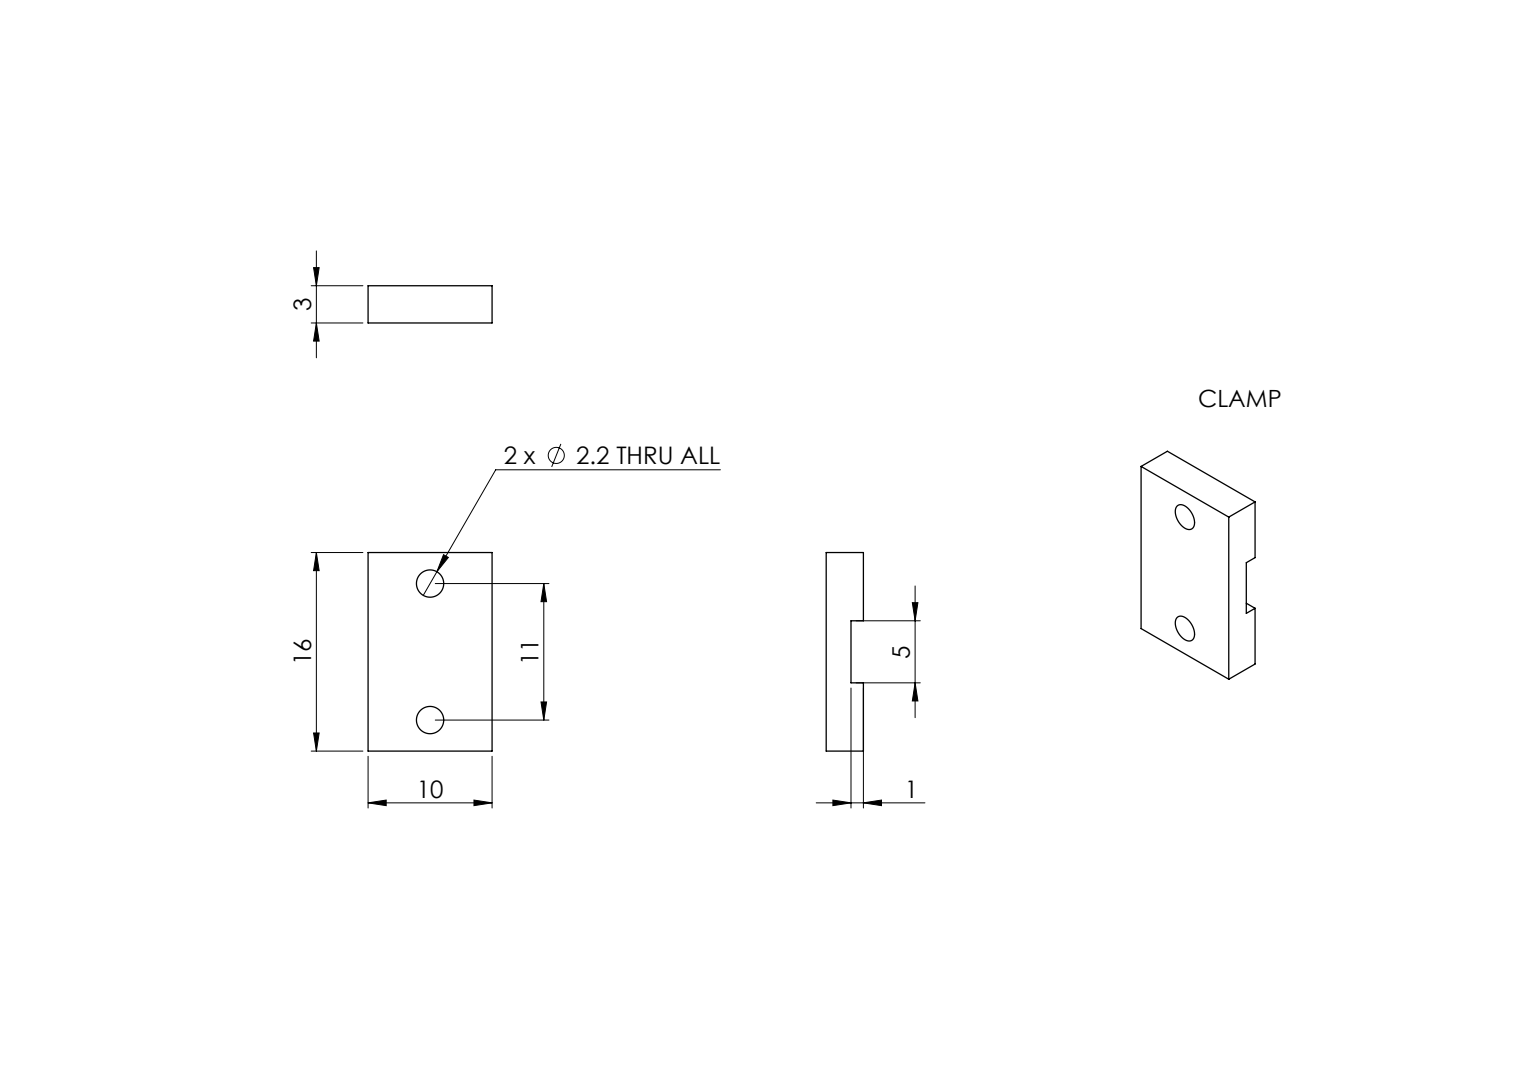
ISO-10303-21;
HEADER;
FILE_DESCRIPTION (('STEP AP214'),
    '1' );
FILE_NAME ('clamp.step',
    '2026-10-27T04:40:18',
    ( '' ),
    ( '' ),
    'SwSTEP 2.0',
    'SolidWorks 2026',
    '' );
FILE_SCHEMA (( 'AUTOMOTIVE_DESIGN' ));
ENDSEC;

DATA;
#33=ORIENTED_EDGE ( 'NONE', *, *, #3045, .T. ) ;
#39=ADVANCED_FACE ( 'NONE', ( #10062, #3972, #586 ), #1625, .F. ) ;
#93=ORIENTED_EDGE ( 'NONE', *, *, #6556, .F. ) ;
#105=CARTESIAN_POINT ( 'NONE',  ( 140.0000000000000284, 8.000000000000000000, 3.000000000000000000 ) ) ;
#116=PLANE ( 'NONE',  #5116 ) ;
#128=ORIENTED_EDGE ( 'NONE', *, *, #1993, .F. ) ;
#135=CARTESIAN_POINT ( 'NONE',  ( -105.0000000000000000, 2.500000000000000000, 4.000000000000000000 ) ) ;
#148=VECTOR ( 'NONE', #1244, 1000.000000000000000 ) ;
#149=ORIENTED_EDGE ( 'NONE', *, *, #772, .F. ) ;
#199=EDGE_LOOP ( 'NONE', ( #1282, #1739, #251, #2267 ) ) ;
#206=CLOSED_SHELL ( 'NONE', ( #8673, #5883, #7933, #4871, #589, #6929, #9618, #1051, #39, #10363, #9693, #7084, #2486, #5406 ) ) ;
#212=AXIS2_PLACEMENT_3D ( 'NONE', #5369, #8063, #3772 ) ;
#233=APPLICATION_CONTEXT ( 'automotive_design' ) ;
#234=VECTOR ( 'NONE', #2072, 1000.000000000000000 ) ;
#244=LINE ( 'NONE', #5283, #6807 ) ;
#251=ORIENTED_EDGE ( 'NONE', *, *, #8511, .F. ) ;
#342=DIRECTION ( 'NONE',  ( 0.000000000000000000, 0.000000000000000000, 1.000000000000000000 ) ) ;
#380=LINE ( 'NONE', #7160, #836 ) ;
#399=PRODUCT_DEFINITION_CONTEXT ( 'detailed design', #1660, 'design' ) ;
#402=CIRCLE ( 'NONE', #212, 1.099999999999989875 ) ;
#445=EDGE_CURVE ( 'NONE', #6076, #9310, #10674, .T. ) ;
#450=ORIENTED_EDGE ( 'NONE', *, *, #772, .T. ) ;
#469=DIRECTION ( 'NONE',  ( 1.000000000000000000, 0.000000000000000000, 0.000000000000000000 ) ) ;
#487=LINE ( 'NONE', #3873, #692 ) ;
#502=ORIENTED_EDGE ( 'NONE', *, *, #6812, .F. ) ;
#511=CARTESIAN_POINT ( 'NONE',  ( 150.0000000000000000, -2.500000000000000444, 6.000000000000000000 ) ) ;
#578=ORIENTED_EDGE ( 'NONE', *, *, #2504, .T. ) ;
#586=FACE_OUTER_BOUND ( 'NONE', #5446, .T. ) ;
#589=ADVANCED_FACE ( 'NONE', ( #5826, #10002 ), #5614, .T. ) ;
#591=VECTOR ( 'NONE', #8546, 1000.000000000000000 ) ;
#651=ORIENTED_EDGE ( 'NONE', *, *, #6556, .T. ) ;
#669=ORIENTED_EDGE ( 'NONE', *, *, #6090, .F. ) ;
#692=VECTOR ( 'NONE', #10647, 1000.000000000000000 ) ;
#702=MECHANICAL_DESIGN_GEOMETRIC_PRESENTATION_REPRESENTATION('',(#1232),#9754);
#743=VECTOR ( 'NONE', #342, 1000.000000000000000 ) ;
#764=CIRCLE ( 'NONE', #5367, 1.099999999999989875 ) ;
#772=EDGE_CURVE ( 'NONE', #7557, #5975, #6044, .T. ) ;
#798=ORIENTED_EDGE ( 'NONE', *, *, #2162, .T. ) ;
#831=DIRECTION ( 'NONE',  ( -0.000000000000000000, 1.000000000000000000, 0.000000000000000000 ) ) ;
#836=VECTOR ( 'NONE', #5537, 1000.000000000000000 ) ;
#847=VERTEX_POINT ( 'NONE', #1713 ) ;
#928=EDGE_CURVE ( 'NONE', #847, #6070, #402, .T. ) ;
#944=CYLINDRICAL_SURFACE ( 'NONE', #4058, 1.099999999999989875 ) ;
#953=ORIENTED_EDGE ( 'NONE', *, *, #8718, .T. ) ;
#970=SURFACE_STYLE_USAGE ( .BOTH. , #1755 ) ;
#979=DIRECTION ( 'NONE',  ( 0.000000000000000000, -0.000000000000000000, -1.000000000000000000 ) ) ;
#983=ORIENTED_EDGE ( 'NONE', *, *, #2088, .F. ) ;
#999=DIRECTION ( 'NONE',  ( -1.000000000000000000, 0.000000000000000000, -0.000000000000000000 ) ) ;
#1017=CYLINDRICAL_SURFACE ( 'NONE', #3505, 1.099999999999989875 ) ;
#1024=FACE_OUTER_BOUND ( 'NONE', #3434, .T. ) ;
#1045=VECTOR ( 'NONE', #1236, 1000.000000000000000 ) ;
#1051=ADVANCED_FACE ( 'NONE', ( #3001 ), #6391, .F. ) ;
#1098=DIRECTION ( 'NONE',  ( 0.000000000000000000, 1.000000000000000000, 0.000000000000000000 ) ) ;
#1126=FACE_OUTER_BOUND ( 'NONE', #4388, .T. ) ;
#1133=ORIENTED_EDGE ( 'NONE', *, *, #1752, .T. ) ;
#1136=VERTEX_POINT ( 'NONE', #5803 ) ;
#1154=EDGE_CURVE ( 'NONE', #5040, #5356, #5860, .T. ) ;
#1226=FACE_OUTER_BOUND ( 'NONE', #5077, .T. ) ;
#1232=STYLED_ITEM ( 'NONE', ( #2645 ), #7886 ) ;
#1236=DIRECTION ( 'NONE',  ( -0.000000000000000000, -0.000000000000000000, 1.000000000000000000 ) ) ;
#1244=DIRECTION ( 'NONE',  ( -1.000000000000000000, 0.000000000000000000, 0.000000000000000000 ) ) ;
#1282=ORIENTED_EDGE ( 'NONE', *, *, #6378, .T. ) ;
#1324=VECTOR ( 'NONE', #9947, 1000.000000000000000 ) ;
#1328=CARTESIAN_POINT ( 'NONE',  ( 143.9000000000000341, 5.500000000000000000, 6.000000000000000000 ) ) ;
#1398=VECTOR ( 'NONE', #3895, 1000.000000000000000 ) ;
#1472=ORIENTED_EDGE ( 'NONE', *, *, #9040, .T. ) ;
#1505=EDGE_LOOP ( 'NONE', ( #10466, #4149, #3036, #8916 ) ) ;
#1508=ORIENTED_EDGE ( 'NONE', *, *, #1752, .F. ) ;
#1522=ORIENTED_EDGE ( 'NONE', *, *, #1154, .F. ) ;
#1556=PRODUCT_DEFINITION_SHAPE ( 'NONE', 'NONE',  #1620 ) ;
#1557=ORIENTED_EDGE ( 'NONE', *, *, #6848, .T. ) ;
#1560=LINE ( 'NONE', #8344, #5022 ) ;
#1594=AXIS2_PLACEMENT_3D ( 'NONE', #1609, #8605, #4362 ) ;
#1609=CARTESIAN_POINT ( 'NONE',  ( 145.0000000000000284, 5.500000000000000000, 6.000000000000000000 ) ) ;
#1620=PRODUCT_DEFINITION ( 'UNKNOWN', '', #6403, #399 ) ;
#1625=PLANE ( 'NONE',  #9971 ) ;
#1648=VERTEX_POINT ( 'NONE', #5161 ) ;
#1660=APPLICATION_CONTEXT ( 'automotive_design' ) ;
#1663=FACE_OUTER_BOUND ( 'NONE', #6726, .T. ) ;
#1706=DIRECTION ( 'NONE',  ( 1.000000000000000000, 0.000000000000000000, 0.000000000000000000 ) ) ;
#1713=CARTESIAN_POINT ( 'NONE',  ( 143.9000000000000341, -5.500000000000000000, 6.000000000000000000 ) ) ;
#1739=ORIENTED_EDGE ( 'NONE', *, *, #7365, .F. ) ;
#1752=EDGE_CURVE ( 'NONE', #1136, #10538, #8935, .T. ) ;
#1755=SURFACE_SIDE_STYLE ('',( #5970 ) ) ;
#1816=DIRECTION ( 'NONE',  ( -0.000000000000000000, -0.000000000000000000, 1.000000000000000000 ) ) ;
#1846=CARTESIAN_POINT ( 'NONE',  ( 146.0999999999999943, -5.500000000000000000, 6.000000000000000000 ) ) ;
#1877=EDGE_CURVE ( 'NONE', #1648, #10538, #7962, .T. ) ;
#1898=ORIENTED_EDGE ( 'NONE', *, *, #3692, .T. ) ;
#1908=STYLED_ITEM('',(#11006),#8465);
#1929=EDGE_CURVE ( 'NONE', #10524, #8381, #2909, .T. ) ;
#1939=EDGE_LOOP ( 'NONE', ( #6034, #3156, #1522, #2323 ) ) ;
#1965=CARTESIAN_POINT ( 'NONE',  ( 150.0000000000000000, 8.000000000000000000, 3.000000000000000000 ) ) ;
#1981=FILL_AREA_STYLE_COLOUR ( '', #9214 ) ;
#1993=EDGE_CURVE ( 'NONE', #10287, #2286, #7346, .T. ) ;
#2045=DIRECTION ( 'NONE',  ( -0.000000000000000000, -1.000000000000000000, -0.000000000000000000 ) ) ;
#2055=CARTESIAN_POINT ( 'NONE',  ( 150.0000000000000000, -8.000000000000000000, 6.000000000000000000 ) ) ;
#2072=DIRECTION ( 'NONE',  ( 1.000000000000000000, -0.000000000000000000, 0.000000000000000000 ) ) ;
#2084=DIRECTION ( 'NONE',  ( -0.000000000000000000, -0.000000000000000000, 1.000000000000000000 ) ) ;
#2088=EDGE_CURVE ( 'NONE', #5975, #8381, #10227, .T. ) ;
#2098=ORIENTED_EDGE ( 'NONE', *, *, #4861, .F. ) ;
#2099=( GEOMETRIC_REPRESENTATION_CONTEXT ( 3 ) GLOBAL_UNCERTAINTY_ASSIGNED_CONTEXT ( ( #7955 ) ) GLOBAL_UNIT_ASSIGNED_CONTEXT ( ( #3880, #2217, #6383 ) ) REPRESENTATION_CONTEXT ( 'NONE', 'WORKASPACE' ) );
#2118=DIRECTION ( 'NONE',  ( -0.000000000000000000, -0.000000000000000000, 1.000000000000000000 ) ) ;
#2129=CARTESIAN_POINT ( 'NONE',  ( 146.0999999999999943, 5.500000000000000000, 6.000000000000000000 ) ) ;
#2130=DIRECTION ( 'NONE',  ( -0.000000000000000000, -0.000000000000000000, 1.000000000000000000 ) ) ;
#2144=AXIS2_PLACEMENT_3D ( 'NONE', #4502, #10617, #3015 ) ;
#2162=EDGE_CURVE ( 'NONE', #9310, #7235, #244, .T. ) ;
#2217=( NAMED_UNIT ( * ) PLANE_ANGLE_UNIT ( ) SI_UNIT ( $, .RADIAN. ) );
#2267=ORIENTED_EDGE ( 'NONE', *, *, #6909, .T. ) ;
#2286=VERTEX_POINT ( 'NONE', #10633 ) ;
#2298=EDGE_CURVE ( 'NONE', #9621, #5032, #764, .T. ) ;
#2307=AXIS2_PLACEMENT_3D ( 'NONE', #5193, #3646, #1706 ) ;
#2319=ORIENTED_EDGE ( 'NONE', *, *, #2298, .F. ) ;
#2323=ORIENTED_EDGE ( 'NONE', *, *, #6378, .F. ) ;
#2368=VECTOR ( 'NONE', #2130, 1000.000000000000000 ) ;
#2383=CARTESIAN_POINT ( 'NONE',  ( 0.000000000000000000, 0.000000000000000000, 3.000000000000000000 ) ) ;
#2412=DIRECTION ( 'NONE',  ( -0.000000000000000000, -1.000000000000000000, -0.000000000000000000 ) ) ;
#2439=DIRECTION ( 'NONE',  ( 0.000000000000000000, 1.000000000000000000, 0.000000000000000000 ) ) ;
#2441=DIRECTION ( 'NONE',  ( 1.000000000000000000, 0.000000000000000000, 0.000000000000000000 ) ) ;
#2464=ORIENTED_EDGE ( 'NONE', *, *, #4239, .T. ) ;
#2466=EDGE_CURVE ( 'NONE', #6070, #847, #10155, .T. ) ;
#2486=ADVANCED_FACE ( 'NONE', ( #5941 ), #6580, .F. ) ;
#2488=ORIENTED_EDGE ( 'NONE', *, *, #6301, .T. ) ;
#2494=CARTESIAN_POINT ( 'NONE',  ( 150.0000000000000000, -8.000000000000000000, 6.000000000000000000 ) ) ;
#2504=EDGE_CURVE ( 'NONE', #10287, #7557, #1560, .T. ) ;
#2512=FACE_BOUND ( 'NONE', #4343, .T. ) ;
#2518=LINE ( 'NONE', #6693, #6429 ) ;
#2549=ORIENTED_EDGE ( 'NONE', *, *, #2298, .T. ) ;
#2566=DIRECTION ( 'NONE',  ( 1.000000000000000000, 0.000000000000000000, 0.000000000000000000 ) ) ;
#2589=CARTESIAN_POINT ( 'NONE',  ( 140.0000000000000284, 8.000000000000000000, 3.000000000000000000 ) ) ;
#2645=PRESENTATION_STYLE_ASSIGNMENT (( #970 ) ) ;
#2715=VECTOR ( 'NONE', #6517, 1000.000000000000000 ) ;
#2751=DIRECTION ( 'NONE',  ( 1.000000000000000000, 0.000000000000000000, 0.000000000000000000 ) ) ;
#2842=CARTESIAN_POINT ( 'NONE',  ( 140.0000000000000568, 2.500000000000000000, 4.000000000000000000 ) ) ;
#2909=LINE ( 'NONE', #6296, #234 ) ;
#2954=CARTESIAN_POINT ( 'NONE',  ( 140.0000000000000284, 2.500000000000000000, 3.000000000000000000 ) ) ;
#2963=LINE ( 'NONE', #2129, #1045 ) ;
#3001=FACE_OUTER_BOUND ( 'NONE', #5813, .T. ) ;
#3003=CARTESIAN_POINT ( 'NONE',  ( 150.0000000000000000, -8.000000000000000000, 6.000000000000000000 ) ) ;
#3015=DIRECTION ( 'NONE',  ( 0.000000000000000000, -0.000000000000000000, 1.000000000000000000 ) ) ;
#3036=ORIENTED_EDGE ( 'NONE', *, *, #7473, .T. ) ;
#3045=EDGE_CURVE ( 'NONE', #9310, #5427, #7645, .T. ) ;
#3121=CARTESIAN_POINT ( 'NONE',  ( 140.0000000000000284, -8.000000000000000000, 6.000000000000000000 ) ) ;
#3156=ORIENTED_EDGE ( 'NONE', *, *, #4861, .T. ) ;
#3176=CARTESIAN_POINT ( 'NONE',  ( 150.0000000000000000, 8.000000000000000000, 6.000000000000000000 ) ) ;
#3217=CARTESIAN_POINT ( 'NONE',  ( 150.0000000000000284, -2.500000000000000000, 4.000000000000000000 ) ) ;
#3319=PLANE ( 'NONE',  #10244 ) ;
#3338=CARTESIAN_POINT ( 'NONE',  ( 0.000000000000000000, 0.000000000000000000, 3.000000000000000000 ) ) ;
#3365=DIRECTION ( 'NONE',  ( 1.000000000000000000, 0.000000000000000000, 0.000000000000000000 ) ) ;
#3409=CARTESIAN_POINT ( 'NONE',  ( 140.0000000000000284, -8.000000000000000000, 3.000000000000000000 ) ) ;
#3427=AXIS2_PLACEMENT_3D ( 'NONE', #5834, #8445, #10785 ) ;
#3434=EDGE_LOOP ( 'NONE', ( #798, #10069, #3716, #5140 ) ) ;
#3469=( LENGTH_UNIT ( ) NAMED_UNIT ( * ) SI_UNIT ( .MILLI., .METRE. ) );
#3474=DIRECTION ( 'NONE',  ( -1.000000000000000000, -0.000000000000000000, -0.000000000000000000 ) ) ;
#3505=AXIS2_PLACEMENT_3D ( 'NONE', #5175, #5124, #2751 ) ;
#3518=AXIS2_PLACEMENT_3D ( 'NONE', #8801, #469, #10626 ) ;
#3554=CARTESIAN_POINT ( 'NONE',  ( 150.0000000000000000, 2.500000000000000000, 3.000000000000000000 ) ) ;
#3557=ORIENTED_EDGE ( 'NONE', *, *, #1877, .F. ) ;
#3588=VECTOR ( 'NONE', #2412, 1000.000000000000000 ) ;
#3597=CARTESIAN_POINT ( 'NONE',  ( 140.0000000000000284, -8.000000000000000000, 6.000000000000000000 ) ) ;
#3634=VERTEX_POINT ( 'NONE', #4108 ) ;
#3646=DIRECTION ( 'NONE',  ( 0.000000000000000000, 0.000000000000000000, 1.000000000000000000 ) ) ;
#3670=CARTESIAN_POINT ( 'NONE',  ( 145.0000000000000284, 5.500000000000000000, 6.000000000000000000 ) ) ;
#3690=ORIENTED_EDGE ( 'NONE', *, *, #928, .F. ) ;
#3692=EDGE_CURVE ( 'NONE', #10524, #3634, #7507, .T. ) ;
#3709=VECTOR ( 'NONE', #5631, 1000.000000000000000 ) ;
#3716=ORIENTED_EDGE ( 'NONE', *, *, #5091, .T. ) ;
#3764=EDGE_CURVE ( 'NONE', #7557, #4954, #5831, .T. ) ;
#3768=AXIS2_PLACEMENT_3D ( 'NONE', #3597, #1098, #6158 ) ;
#3772=DIRECTION ( 'NONE',  ( 1.000000000000000000, 0.000000000000000000, 0.000000000000000000 ) ) ;
#3819=SHAPE_REPRESENTATION_RELATIONSHIP ( 'NONE' , 'NONE' ,  #10405, #7886 ) ;
#3832=ORIENTED_EDGE ( 'NONE', *, *, #928, .T. ) ;
#3873=CARTESIAN_POINT ( 'NONE',  ( 150.0000000000000000, -8.000000000000000000, 3.000000000000000000 ) ) ;
#3876=ORIENTED_EDGE ( 'NONE', *, *, #7132, .T. ) ;
#3880=( LENGTH_UNIT ( ) NAMED_UNIT ( * ) SI_UNIT ( .MILLI., .METRE. ) );
#3895=DIRECTION ( 'NONE',  ( 0.000000000000000000, 0.000000000000000000, -1.000000000000000000 ) ) ;
#3903=LINE ( 'NONE', #7294, #6212 ) ;
#3972=FACE_BOUND ( 'NONE', #5458, .T. ) ;
#4007=DIRECTION ( 'NONE',  ( 0.000000000000000000, 0.000000000000000000, 1.000000000000000000 ) ) ;
#4058=AXIS2_PLACEMENT_3D ( 'NONE', #9334, #7732, #8404 ) ;
#4071=VECTOR ( 'NONE', #2045, 1000.000000000000000 ) ;
#4095=DIRECTION ( 'NONE',  ( -1.000000000000000000, 0.000000000000000000, 0.000000000000000000 ) ) ;
#4108=CARTESIAN_POINT ( 'NONE',  ( 140.0000000000000568, -2.500000000000000000, 4.000000000000000000 ) ) ;
#4132=EDGE_LOOP ( 'NONE', ( #5405, #2319, #1557, #4656 ) ) ;
#4149=ORIENTED_EDGE ( 'NONE', *, *, #1877, .T. ) ;
#4228=ORIENTED_EDGE ( 'NONE', *, *, #5091, .F. ) ;
#4239=EDGE_CURVE ( 'NONE', #5427, #5356, #9469, .T. ) ;
#4246=DIRECTION ( 'NONE',  ( -0.000000000000000000, -0.000000000000000000, 1.000000000000000000 ) ) ;
#4272=CARTESIAN_POINT ( 'NONE',  ( 150.0000000000000000, 8.000000000000000000, 6.000000000000000000 ) ) ;
#4284=DIRECTION ( 'NONE',  ( 0.000000000000000000, -1.000000000000000000, 0.000000000000000000 ) ) ;
#4327=DIRECTION ( 'NONE',  ( -0.000000000000000000, -0.000000000000000000, -1.000000000000000000 ) ) ;
#4343=EDGE_LOOP ( 'NONE', ( #2549, #2488 ) ) ;
#4346=( LENGTH_UNIT ( ) NAMED_UNIT ( * ) SI_UNIT ( .MILLI., .METRE. ) );
#4362=DIRECTION ( 'NONE',  ( 1.000000000000000000, 0.000000000000000000, 0.000000000000000000 ) ) ;
#4369=CARTESIAN_POINT ( 'NONE',  ( 140.0000000000000284, -8.000000000000000000, 4.000000000000000000 ) ) ;
#4388=EDGE_LOOP ( 'NONE', ( #4659, #4228, #5013, #651, #128, #502, #8779, #5188 ) ) ;
#4396=AXIS2_PLACEMENT_3D ( 'NONE', #4668, #4825, #8181 ) ;
#4414=LINE ( 'NONE', #5357, #4071 ) ;
#4472=VECTOR ( 'NONE', #4007, 1000.000000000000000 ) ;
#4480=EDGE_LOOP ( 'NONE', ( #6392, #5597, #10932, #8542, #450, #8676, #5228, #8441 ) ) ;
#4492=CARTESIAN_POINT ( 'NONE',  ( 145.0000000000000284, 5.500000000000000000, 6.000000000000000000 ) ) ;
#4502=CARTESIAN_POINT ( 'NONE',  ( -105.0000000000000000, -2.500000000000000000, 4.000000000000000000 ) ) ;
#4572=ORIENTED_EDGE ( 'NONE', *, *, #7473, .F. ) ;
#4582=CARTESIAN_POINT ( 'NONE',  ( 0.000000000000000000, 0.000000000000000000, 4.000000000000000000 ) ) ;
#4592=AXIS2_PLACEMENT_3D ( 'NONE', #6820, #4246, #3365 ) ;
#4608=CARTESIAN_POINT ( 'NONE',  ( 150.0000000000000284, 2.500000000000000000, 4.000000000000000000 ) ) ;
#4656=ORIENTED_EDGE ( 'NONE', *, *, #2466, .T. ) ;
#4658=EDGE_CURVE ( 'NONE', #3634, #7235, #2518, .T. ) ;
#4659=ORIENTED_EDGE ( 'NONE', *, *, #4239, .F. ) ;
#4668=CARTESIAN_POINT ( 'NONE',  ( 145.0000000000000284, 5.500000000000000000, 3.000000000000000888 ) ) ;
#4671=ORIENTED_EDGE ( 'NONE', *, *, #8511, .T. ) ;
#4681=ORIENTED_EDGE ( 'NONE', *, *, #445, .T. ) ;
#4684=PRODUCT_CONTEXT ( 'NONE', #233, 'mechanical' ) ;
#4702=CARTESIAN_POINT ( 'NONE',  ( 150.0000000000000000, -2.500000000000000444, 3.000000000000000000 ) ) ;
#4775=CIRCLE ( 'NONE', #9761, 1.099999999999989875 ) ;
#4795=ORIENTED_EDGE ( 'NONE', *, *, #1929, .F. ) ;
#4818=PLANE ( 'NONE',  #8701 ) ;
#4825=DIRECTION ( 'NONE',  ( -0.000000000000000000, -0.000000000000000000, 1.000000000000000000 ) ) ;
#4861=EDGE_CURVE ( 'NONE', #6076, #5356, #7074, .T. ) ;
#4871=ADVANCED_FACE ( 'NONE', ( #1126 ), #9800, .F. ) ;
#4942=CARTESIAN_POINT ( 'NONE',  ( 145.0000000000000284, -5.500000000000000000, 6.000000000000000000 ) ) ;
#4954=VERTEX_POINT ( 'NONE', #3176 ) ;
#4987=ORIENTED_EDGE ( 'NONE', *, *, #1929, .T. ) ;
#5000=FACE_OUTER_BOUND ( 'NONE', #6134, .T. ) ;
#5013=ORIENTED_EDGE ( 'NONE', *, *, #3692, .F. ) ;
#5022=VECTOR ( 'NONE', #6677, 1000.000000000000000 ) ;
#5032=VERTEX_POINT ( 'NONE', #7510 ) ;
#5040=VERTEX_POINT ( 'NONE', #105 ) ;
#5077=EDGE_LOOP ( 'NONE', ( #3557, #669, #3876, #1133 ) ) ;
#5091=EDGE_CURVE ( 'NONE', #3634, #5427, #5889, .T. ) ;
#5116=AXIS2_PLACEMENT_3D ( 'NONE', #3338, #5269, #999 ) ;
#5118=CARTESIAN_POINT ( 'NONE',  ( 150.0000000000000000, -8.000000000000000000, 3.000000000000000000 ) ) ;
#5124=DIRECTION ( 'NONE',  ( -0.000000000000000000, -0.000000000000000000, 1.000000000000000000 ) ) ;
#5140=ORIENTED_EDGE ( 'NONE', *, *, #3045, .F. ) ;
#5159=ORIENTED_EDGE ( 'NONE', *, *, #1993, .T. ) ;
#5161=CARTESIAN_POINT ( 'NONE',  ( 143.9000000000000341, 5.500000000000000000, 3.000000000000000888 ) ) ;
#5175=CARTESIAN_POINT ( 'NONE',  ( 145.0000000000000284, 5.500000000000000000, 6.000000000000000000 ) ) ;
#5182=( NAMED_UNIT ( * ) PLANE_ANGLE_UNIT ( ) SI_UNIT ( $, .RADIAN. ) );
#5188=ORIENTED_EDGE ( 'NONE', *, *, #1154, .T. ) ;
#5193=CARTESIAN_POINT ( 'NONE',  ( 0.000000000000000000, 0.000000000000000000, 0.000000000000000000 ) ) ;
#5216=EDGE_LOOP ( 'NONE', ( #1508, #4572 ) ) ;
#5228=ORIENTED_EDGE ( 'NONE', *, *, #5376, .F. ) ;
#5239=( NAMED_UNIT ( * ) SI_UNIT ( $, .STERADIAN. ) SOLID_ANGLE_UNIT ( ) );
#5269=DIRECTION ( 'NONE',  ( 0.000000000000000000, 0.000000000000000000, -1.000000000000000000 ) ) ;
#5283=CARTESIAN_POINT ( 'NONE',  ( 150.0000000000000000, -8.000000000000000000, 4.000000000000000000 ) ) ;
#5289=LINE ( 'NONE', #3409, #9909 ) ;
#5296=DIRECTION ( 'NONE',  ( 0.000000000000000000, 0.000000000000000000, -1.000000000000000000 ) ) ;
#5340=DIRECTION ( 'NONE',  ( 0.000000000000000000, 1.000000000000000000, 0.000000000000000000 ) ) ;
#5351=FILL_AREA_STYLE ('',( #1981 ) ) ;
#5353=AXIS2_PLACEMENT_3D ( 'NONE', #2383, #10776, #7397 ) ;
#5356=VERTEX_POINT ( 'NONE', #2954 ) ;
#5357=CARTESIAN_POINT ( 'NONE',  ( 140.0000000000000284, -8.000000000000000000, 3.000000000000000000 ) ) ;
#5367=AXIS2_PLACEMENT_3D ( 'NONE', #5401, #2084, #8977 ) ;
#5369=CARTESIAN_POINT ( 'NONE',  ( 145.0000000000000284, -5.500000000000000000, 6.000000000000000000 ) ) ;
#5376=EDGE_CURVE ( 'NONE', #7235, #8381, #5379, .T. ) ;
#5379=LINE ( 'NONE', #511, #1398 ) ;
#5385=CARTESIAN_POINT ( 'NONE',  ( 146.0999999999999943, -5.500000000000000000, 6.000000000000000000 ) ) ;
#5401=CARTESIAN_POINT ( 'NONE',  ( 145.0000000000000284, -5.500000000000000000, 3.000000000000000888 ) ) ;
#5405=ORIENTED_EDGE ( 'NONE', *, *, #9040, .F. ) ;
#5406=ADVANCED_FACE ( 'NONE', ( #1226 ), #8728, .F. ) ;
#5427=VERTEX_POINT ( 'NONE', #2842 ) ;
#5446=EDGE_LOOP ( 'NONE', ( #7439, #4671, #8814, #578 ) ) ;
#5458=EDGE_LOOP ( 'NONE', ( #8088, #3690 ) ) ;
#5473=ORIENTED_EDGE ( 'NONE', *, *, #8718, .F. ) ;
#5537=DIRECTION ( 'NONE',  ( -1.000000000000000000, -0.000000000000000000, -0.000000000000000000 ) ) ;
#5597=ORIENTED_EDGE ( 'NONE', *, *, #10656, .T. ) ;
#5614=PLANE ( 'NONE',  #5353 ) ;
#5631=DIRECTION ( 'NONE',  ( -0.000000000000000000, -1.000000000000000000, -0.000000000000000000 ) ) ;
#5803=CARTESIAN_POINT ( 'NONE',  ( 146.0999999999999943, 5.500000000000000000, 6.000000000000000000 ) ) ;
#5813=EDGE_LOOP ( 'NONE', ( #953, #149, #10092, #5159 ) ) ;
#5826=FACE_BOUND ( 'NONE', #10967, .T. ) ;
#5831=LINE ( 'NONE', #10051, #10140 ) ;
#5834=CARTESIAN_POINT ( 'NONE',  ( 145.0000000000000284, -5.500000000000000000, 6.000000000000000000 ) ) ;
#5860=LINE ( 'NONE', #10863, #3588 ) ;
#5876=CARTESIAN_POINT ( 'NONE',  ( 146.0999999999999943, -5.500000000000000000, 3.000000000000000888 ) ) ;
#5883=ADVANCED_FACE ( 'NONE', ( #5000 ), #944, .F. ) ;
#5889=LINE ( 'NONE', #4369, #9739 ) ;
#5941=FACE_OUTER_BOUND ( 'NONE', #4132, .T. ) ;
#5970=SURFACE_STYLE_FILL_AREA ( #5351 ) ;
#5971=CARTESIAN_POINT ( 'NONE',  ( 140.0000000000000284, -8.000000000000000000, 6.000000000000000000 ) ) ;
#5975=VERTEX_POINT ( 'NONE', #9675 ) ;
#6012=( GEOMETRIC_REPRESENTATION_CONTEXT ( 3 ) GLOBAL_UNCERTAINTY_ASSIGNED_CONTEXT ( ( #8850 ) ) GLOBAL_UNIT_ASSIGNED_CONTEXT ( ( #3469, #5182, #6087 ) ) REPRESENTATION_CONTEXT ( 'NONE', 'WORKASPACE' ) );
#6034=ORIENTED_EDGE ( 'NONE', *, *, #10656, .F. ) ;
#6044=LINE ( 'NONE', #2494, #591 ) ;
#6070=VERTEX_POINT ( 'NONE', #5385 ) ;
#6076=VERTEX_POINT ( 'NONE', #3554 ) ;
#6087=( NAMED_UNIT ( * ) SI_UNIT ( $, .STERADIAN. ) SOLID_ANGLE_UNIT ( ) );
#6090=EDGE_CURVE ( 'NONE', #9455, #1648, #10441, .T. ) ;
#6134=EDGE_LOOP ( 'NONE', ( #10605, #1472, #3832, #6703 ) ) ;
#6158=DIRECTION ( 'NONE',  ( 0.000000000000000000, -0.000000000000000000, 1.000000000000000000 ) ) ;
#6212=VECTOR ( 'NONE', #10679, 1000.000000000000000 ) ;
#6295=PLANE ( 'NONE',  #2144 ) ;
#6296=CARTESIAN_POINT ( 'NONE',  ( -0.000000000000000000, -2.500000000000000000, 3.000000000000000000 ) ) ;
#6301=EDGE_CURVE ( 'NONE', #5032, #9621, #9374, .T. ) ;
#6325=LINE ( 'NONE', #9708, #3709 ) ;
#6378=EDGE_CURVE ( 'NONE', #8797, #5040, #9311, .T. ) ;
#6383=( NAMED_UNIT ( * ) SI_UNIT ( $, .STERADIAN. ) SOLID_ANGLE_UNIT ( ) );
#6391=PLANE ( 'NONE',  #3768 ) ;
#6392=ORIENTED_EDGE ( 'NONE', *, *, #445, .F. ) ;
#6398=CIRCLE ( 'NONE', #1594, 1.099999999999989875 ) ;
#6403=PRODUCT_DEFINITION_FORMATION_WITH_SPECIFIED_SOURCE ( 'ANY', '', #9011, .NOT_KNOWN. ) ;
#6409=FACE_OUTER_BOUND ( 'NONE', #8808, .T. ) ;
#6410=UNCERTAINTY_MEASURE_WITH_UNIT (LENGTH_MEASURE( 1.000000000000000082E-05 ), #4346, 'distance_accuracy_value', 'NONE');
#6429=VECTOR ( 'NONE', #9247, 1000.000000000000000 ) ;
#6463=EDGE_CURVE ( 'NONE', #1648, #9455, #4775, .T. ) ;
#6471=CARTESIAN_POINT ( 'NONE',  ( 140.0000000000000284, -2.500000000000000444, 6.000000000000000000 ) ) ;
#6517=DIRECTION ( 'NONE',  ( -0.000000000000000000, -0.000000000000000000, -1.000000000000000000 ) ) ;
#6556=EDGE_CURVE ( 'NONE', #10524, #2286, #4414, .T. ) ;
#6580=CYLINDRICAL_SURFACE ( 'NONE', #10348, 1.099999999999989875 ) ;
#6583=LINE ( 'NONE', #7354, #8844 ) ;
#6589=CARTESIAN_POINT ( 'NONE',  ( 0.000000000000000000, 0.000000000000000000, 6.000000000000000000 ) ) ;
#6677=DIRECTION ( 'NONE',  ( 1.000000000000000000, 0.000000000000000000, 0.000000000000000000 ) ) ;
#6693=CARTESIAN_POINT ( 'NONE',  ( -105.0000000000000000, -2.500000000000000000, 4.000000000000000000 ) ) ;
#6703=ORIENTED_EDGE ( 'NONE', *, *, #6848, .F. ) ;
#6713=VERTEX_POINT ( 'NONE', #10018 ) ;
#6726=EDGE_LOOP ( 'NONE', ( #4681, #33, #2464, #2098 ) ) ;
#6807=VECTOR ( 'NONE', #4284, 1000.000000000000000 ) ;
#6812=EDGE_CURVE ( 'NONE', #6713, #10287, #6325, .T. ) ;
#6820=CARTESIAN_POINT ( 'NONE',  ( 145.0000000000000284, -5.500000000000000000, 3.000000000000000888 ) ) ;
#6848=EDGE_CURVE ( 'NONE', #9621, #6070, #10114, .T. ) ;
#6878=FACE_OUTER_BOUND ( 'NONE', #199, .T. ) ;
#6903=DIRECTION ( 'NONE',  ( -0.000000000000000000, -0.000000000000000000, 1.000000000000000000 ) ) ;
#6909=EDGE_CURVE ( 'NONE', #4954, #8797, #9338, .T. ) ;
#6923=CARTESIAN_POINT ( 'NONE',  ( 140.0000000000000284, 2.500000000000000444, 6.000000000000000000 ) ) ;
#6927=( NAMED_UNIT ( * ) PLANE_ANGLE_UNIT ( ) SI_UNIT ( $, .RADIAN. ) );
#6929=ADVANCED_FACE ( 'NONE', ( #2512, #10217 ), #116, .T. ) ;
#6971=AXIS2_PLACEMENT_3D ( 'NONE', #3670, #10169, #2566 ) ;
#7074=LINE ( 'NONE', #9629, #148 ) ;
#7084=ADVANCED_FACE ( 'NONE', ( #6409 ), #6295, .T. ) ;
#7132=EDGE_CURVE ( 'NONE', #9455, #1136, #2963, .T. ) ;
#7157=DIRECTION ( 'NONE',  ( 1.000000000000000000, 0.000000000000000000, 0.000000000000000000 ) ) ;
#7160=CARTESIAN_POINT ( 'NONE',  ( 140.0000000000000284, 8.000000000000000000, 6.000000000000000000 ) ) ;
#7235=VERTEX_POINT ( 'NONE', #3217 ) ;
#7247=SHAPE_DEFINITION_REPRESENTATION ( #1556, #10405 ) ;
#7294=CARTESIAN_POINT ( 'NONE',  ( 140.0000000000000284, 8.000000000000000000, 6.000000000000000000 ) ) ;
#7346=LINE ( 'NONE', #3121, #2715 ) ;
#7354=CARTESIAN_POINT ( 'NONE',  ( 143.9000000000000341, -5.500000000000000000, 6.000000000000000000 ) ) ;
#7361=DIRECTION ( 'NONE',  ( 0.000000000000000000, 0.000000000000000000, -1.000000000000000000 ) ) ;
#7365=EDGE_CURVE ( 'NONE', #6713, #5040, #3903, .T. ) ;
#7397=DIRECTION ( 'NONE',  ( -1.000000000000000000, 0.000000000000000000, -0.000000000000000000 ) ) ;
#7439=ORIENTED_EDGE ( 'NONE', *, *, #3764, .T. ) ;
#7473=EDGE_CURVE ( 'NONE', #10538, #1136, #6398, .T. ) ;
#7490=DIRECTION ( 'NONE',  ( 0.000000000000000000, 0.000000000000000000, 1.000000000000000000 ) ) ;
#7507=LINE ( 'NONE', #6471, #4472 ) ;
#7510=CARTESIAN_POINT ( 'NONE',  ( 143.9000000000000341, -5.500000000000000000, 3.000000000000000888 ) ) ;
#7557=VERTEX_POINT ( 'NONE', #2055 ) ;
#7604=DIRECTION ( 'NONE',  ( 0.000000000000000000, -0.000000000000000000, -1.000000000000000000 ) ) ;
#7645=LINE ( 'NONE', #135, #1324 ) ;
#7732=DIRECTION ( 'NONE',  ( -0.000000000000000000, -0.000000000000000000, 1.000000000000000000 ) ) ;
#7752=DIRECTION ( 'NONE',  ( 1.000000000000000000, 0.000000000000000000, 0.000000000000000000 ) ) ;
#7803=VECTOR ( 'NONE', #3474, 1000.000000000000000 ) ;
#7830=VECTOR ( 'NONE', #9412, 1000.000000000000000 ) ;
#7886=ADVANCED_BREP_SHAPE_REPRESENTATION ( '', ( #8465, #2307 ), #6012 ) ;
#7933=ADVANCED_FACE ( 'NONE', ( #9157 ), #4818, .F. ) ;
#7955=UNCERTAINTY_MEASURE_WITH_UNIT (LENGTH_MEASURE( 1.000000000000000082E-05 ), #3880, 'distance_accuracy_value', 'NONE');
#7962=LINE ( 'NONE', #9623, #2368 ) ;
#8063=DIRECTION ( 'NONE',  ( -0.000000000000000000, -0.000000000000000000, 1.000000000000000000 ) ) ;
#8088=ORIENTED_EDGE ( 'NONE', *, *, #2466, .F. ) ;
#8131=MECHANICAL_DESIGN_GEOMETRIC_PRESENTATION_REPRESENTATION('',(#1908),#2099);
#8150=AXIS2_PLACEMENT_3D ( 'NONE', #4492, #2118, #8785 ) ;
#8181=DIRECTION ( 'NONE',  ( 1.000000000000000000, 0.000000000000000000, 0.000000000000000000 ) ) ;
#8193=ORIENTED_EDGE ( 'NONE', *, *, #6090, .T. ) ;
#8284=ORIENTED_EDGE ( 'NONE', *, *, #6463, .T. ) ;
#8344=CARTESIAN_POINT ( 'NONE',  ( 140.0000000000000284, -8.000000000000000000, 6.000000000000000000 ) ) ;
#8347=DIRECTION ( 'NONE',  ( -0.000000000000000000, -0.000000000000000000, 1.000000000000000000 ) ) ;
#8381=VERTEX_POINT ( 'NONE', #4702 ) ;
#8404=DIRECTION ( 'NONE',  ( 1.000000000000000000, 0.000000000000000000, 0.000000000000000000 ) ) ;
#8435=CARTESIAN_POINT ( 'NONE',  ( -105.0000000000000000, 2.500000000000000000, 4.000000000000000000 ) ) ;
#8441=ORIENTED_EDGE ( 'NONE', *, *, #2162, .F. ) ;
#8445=DIRECTION ( 'NONE',  ( -0.000000000000000000, -0.000000000000000000, 1.000000000000000000 ) ) ;
#8465=MANIFOLD_SOLID_BREP ( 'M2 Clearance Hole1', #206 ) ;
#8511=EDGE_CURVE ( 'NONE', #4954, #6713, #380, .T. ) ;
#8542=ORIENTED_EDGE ( 'NONE', *, *, #3764, .F. ) ;
#8546=DIRECTION ( 'NONE',  ( -0.000000000000000000, -0.000000000000000000, -1.000000000000000000 ) ) ;
#8605=DIRECTION ( 'NONE',  ( -0.000000000000000000, -0.000000000000000000, 1.000000000000000000 ) ) ;
#8647=CARTESIAN_POINT ( 'NONE',  ( 145.0000000000000284, 5.500000000000000000, 3.000000000000000888 ) ) ;
#8673=ADVANCED_FACE ( 'NONE', ( #9522 ), #1017, .F. ) ;
#8676=ORIENTED_EDGE ( 'NONE', *, *, #2088, .T. ) ;
#8701=AXIS2_PLACEMENT_3D ( 'NONE', #3003, #4095, #7490 ) ;
#8718=EDGE_CURVE ( 'NONE', #2286, #5975, #5289, .T. ) ;
#8728=CYLINDRICAL_SURFACE ( 'NONE', #8150, 1.099999999999989875 ) ;
#8735=CARTESIAN_POINT ( 'NONE',  ( 150.0000000000000000, 2.500000000000000444, 6.000000000000000000 ) ) ;
#8765=DIRECTION ( 'NONE',  ( -1.000000000000000000, 0.000000000000000000, -0.000000000000000000 ) ) ;
#8779=ORIENTED_EDGE ( 'NONE', *, *, #7365, .T. ) ;
#8785=DIRECTION ( 'NONE',  ( 1.000000000000000000, 0.000000000000000000, 0.000000000000000000 ) ) ;
#8797=VERTEX_POINT ( 'NONE', #1965 ) ;
#8801=CARTESIAN_POINT ( 'NONE',  ( 140.0000000000000284, -8.000000000000000000, 6.000000000000000000 ) ) ;
#8808=EDGE_LOOP ( 'NONE', ( #10586, #4795, #1898, #10849 ) ) ;
#8814=ORIENTED_EDGE ( 'NONE', *, *, #6812, .T. ) ;
#8844=VECTOR ( 'NONE', #8347, 1000.000000000000000 ) ;
#8850=UNCERTAINTY_MEASURE_WITH_UNIT (LENGTH_MEASURE( 1.000000000000000082E-05 ), #3469, 'distance_accuracy_value', 'NONE');
#8916=ORIENTED_EDGE ( 'NONE', *, *, #7132, .F. ) ;
#8935=CIRCLE ( 'NONE', #6971, 1.099999999999989875 ) ;
#8977=DIRECTION ( 'NONE',  ( 1.000000000000000000, 0.000000000000000000, 0.000000000000000000 ) ) ;
#9011=PRODUCT ( 'clamp', 'clamp', '', ( #4684 ) ) ;
#9040=EDGE_CURVE ( 'NONE', #5032, #847, #6583, .T. ) ;
#9157=FACE_OUTER_BOUND ( 'NONE', #4480, .T. ) ;
#9173=DIRECTION ( 'NONE',  ( -0.000000000000000000, -0.000000000000000000, 1.000000000000000000 ) ) ;
#9214=COLOUR_RGB ( '',0.8941176470588234615, 0.8941176470588234615, 0.8941176470588234615 ) ;
#9247=DIRECTION ( 'NONE',  ( 1.000000000000000000, 0.000000000000000000, 0.000000000000000000 ) ) ;
#9310=VERTEX_POINT ( 'NONE', #4608 ) ;
#9311=LINE ( 'NONE', #2589, #7803 ) ;
#9334=CARTESIAN_POINT ( 'NONE',  ( 145.0000000000000284, -5.500000000000000000, 6.000000000000000000 ) ) ;
#9338=LINE ( 'NONE', #4272, #9933 ) ;
#9374=CIRCLE ( 'NONE', #4592, 1.099999999999989875 ) ;
#9382=VECTOR ( 'NONE', #6903, 1000.000000000000000 ) ;
#9412=DIRECTION ( 'NONE',  ( 0.000000000000000000, 0.000000000000000000, -1.000000000000000000 ) ) ;
#9455=VERTEX_POINT ( 'NONE', #10499 ) ;
#9469=LINE ( 'NONE', #6923, #7830 ) ;
#9522=FACE_OUTER_BOUND ( 'NONE', #1505, .T. ) ;
#9548=AXIS2_PLACEMENT_3D ( 'NONE', #10929, #10094, #7604 ) ;
#9561=AXIS2_PLACEMENT_3D ( 'NONE', #4582, #5296, #8765 ) ;
#9618=ADVANCED_FACE ( 'NONE', ( #6878 ), #10881, .F. ) ;
#9621=VERTEX_POINT ( 'NONE', #5876 ) ;
#9623=CARTESIAN_POINT ( 'NONE',  ( 143.9000000000000341, 5.500000000000000000, 6.000000000000000000 ) ) ;
#9629=CARTESIAN_POINT ( 'NONE',  ( 0.000000000000000000, 2.500000000000000000, 3.000000000000000000 ) ) ;
#9675=CARTESIAN_POINT ( 'NONE',  ( 150.0000000000000000, -8.000000000000000000, 3.000000000000000000 ) ) ;
#9693=ADVANCED_FACE ( 'NONE', ( #1663 ), #3319, .T. ) ;
#9708=CARTESIAN_POINT ( 'NONE',  ( 140.0000000000000284, -8.000000000000000000, 6.000000000000000000 ) ) ;
#9739=VECTOR ( 'NONE', #831, 1000.000000000000000 ) ;
#9754=( GEOMETRIC_REPRESENTATION_CONTEXT ( 3 ) GLOBAL_UNCERTAINTY_ASSIGNED_CONTEXT ( ( #6410 ) ) GLOBAL_UNIT_ASSIGNED_CONTEXT ( ( #4346, #6927, #5239 ) ) REPRESENTATION_CONTEXT ( 'NONE', 'WORKASPACE' ) );
#9761=AXIS2_PLACEMENT_3D ( 'NONE', #8647, #1816, #7157 ) ;
#9800=PLANE ( 'NONE',  #3518 ) ;
#9909=VECTOR ( 'NONE', #7752, 1000.000000000000000 ) ;
#9933=VECTOR ( 'NONE', #4327, 1000.000000000000000 ) ;
#9947=DIRECTION ( 'NONE',  ( -1.000000000000000000, -0.000000000000000000, -0.000000000000000000 ) ) ;
#9971=AXIS2_PLACEMENT_3D ( 'NONE', #6589, #7361, #10746 ) ;
#9998=VECTOR ( 'NONE', #5340, 1000.000000000000000 ) ;
#10002=FACE_OUTER_BOUND ( 'NONE', #1939, .T. ) ;
#10018=CARTESIAN_POINT ( 'NONE',  ( 140.0000000000000284, 8.000000000000000000, 6.000000000000000000 ) ) ;
#10051=CARTESIAN_POINT ( 'NONE',  ( 150.0000000000000000, -8.000000000000000000, 6.000000000000000000 ) ) ;
#10062=FACE_BOUND ( 'NONE', #5216, .T. ) ;
#10069=ORIENTED_EDGE ( 'NONE', *, *, #4658, .F. ) ;
#10092=ORIENTED_EDGE ( 'NONE', *, *, #2504, .F. ) ;
#10094=DIRECTION ( 'NONE',  ( 0.000000000000000000, -1.000000000000000000, 0.000000000000000000 ) ) ;
#10114=LINE ( 'NONE', #1846, #9382 ) ;
#10140=VECTOR ( 'NONE', #2439, 1000.000000000000000 ) ;
#10145=DIRECTION ( 'NONE',  ( 0.000000000000000000, -1.000000000000000000, 0.000000000000000000 ) ) ;
#10155=CIRCLE ( 'NONE', #3427, 1.099999999999989875 ) ;
#10169=DIRECTION ( 'NONE',  ( -0.000000000000000000, -0.000000000000000000, 1.000000000000000000 ) ) ;
#10217=FACE_OUTER_BOUND ( 'NONE', #10344, .T. ) ;
#10227=LINE ( 'NONE', #5118, #9998 ) ;
#10244=AXIS2_PLACEMENT_3D ( 'NONE', #8435, #10145, #979 ) ;
#10287=VERTEX_POINT ( 'NONE', #5971 ) ;
#10344=EDGE_LOOP ( 'NONE', ( #93, #4987, #983, #5473 ) ) ;
#10348=AXIS2_PLACEMENT_3D ( 'NONE', #4942, #9173, #2441 ) ;
#10363=ADVANCED_FACE ( 'NONE', ( #1024 ), #10414, .T. ) ;
#10405=SHAPE_REPRESENTATION ( 'clamp', ( #2307 ), #6012 ) ;
#10414=PLANE ( 'NONE',  #9561 ) ;
#10441=CIRCLE ( 'NONE', #4396, 1.099999999999989875 ) ;
#10466=ORIENTED_EDGE ( 'NONE', *, *, #6463, .F. ) ;
#10499=CARTESIAN_POINT ( 'NONE',  ( 146.0999999999999943, 5.500000000000000000, 3.000000000000000888 ) ) ;
#10524=VERTEX_POINT ( 'NONE', #10897 ) ;
#10538=VERTEX_POINT ( 'NONE', #1328 ) ;
#10586=ORIENTED_EDGE ( 'NONE', *, *, #5376, .T. ) ;
#10605=ORIENTED_EDGE ( 'NONE', *, *, #6301, .F. ) ;
#10617=DIRECTION ( 'NONE',  ( 0.000000000000000000, 1.000000000000000000, 0.000000000000000000 ) ) ;
#10626=DIRECTION ( 'NONE',  ( 0.000000000000000000, 0.000000000000000000, -1.000000000000000000 ) ) ;
#10633=CARTESIAN_POINT ( 'NONE',  ( 140.0000000000000284, -8.000000000000000000, 3.000000000000000000 ) ) ;
#10647=DIRECTION ( 'NONE',  ( 0.000000000000000000, 1.000000000000000000, 0.000000000000000000 ) ) ;
#10656=EDGE_CURVE ( 'NONE', #6076, #8797, #487, .T. ) ;
#10674=LINE ( 'NONE', #8735, #743 ) ;
#10679=DIRECTION ( 'NONE',  ( -0.000000000000000000, -0.000000000000000000, -1.000000000000000000 ) ) ;
#10746=DIRECTION ( 'NONE',  ( -1.000000000000000000, 0.000000000000000000, -0.000000000000000000 ) ) ;
#10776=DIRECTION ( 'NONE',  ( 0.000000000000000000, 0.000000000000000000, -1.000000000000000000 ) ) ;
#10785=DIRECTION ( 'NONE',  ( 1.000000000000000000, 0.000000000000000000, 0.000000000000000000 ) ) ;
#10849=ORIENTED_EDGE ( 'NONE', *, *, #4658, .T. ) ;
#10863=CARTESIAN_POINT ( 'NONE',  ( 140.0000000000000284, -8.000000000000000000, 3.000000000000000000 ) ) ;
#10881=PLANE ( 'NONE',  #9548 ) ;
#10897=CARTESIAN_POINT ( 'NONE',  ( 140.0000000000000284, -2.500000000000000000, 3.000000000000000000 ) ) ;
#10929=CARTESIAN_POINT ( 'NONE',  ( 140.0000000000000284, 8.000000000000000000, 6.000000000000000000 ) ) ;
#10932=ORIENTED_EDGE ( 'NONE', *, *, #6909, .F. ) ;
#10967=EDGE_LOOP ( 'NONE', ( #8193, #8284 ) ) ;
#11000=COLOUR_RGB('Light Blue',0.38,0.62,0.78);
#11001=FILL_AREA_STYLE_COLOUR('',#11000);
#11002=FILL_AREA_STYLE('',(#11001));
#11003=SURFACE_STYLE_FILL_AREA(#11002);
#11004=SURFACE_SIDE_STYLE('',(#11003));
#11005=SURFACE_STYLE_USAGE(.BOTH.,#11004);
#11006=PRESENTATION_STYLE_ASSIGNMENT((#11005));
ENDSEC;
END-ISO-10303-21;
